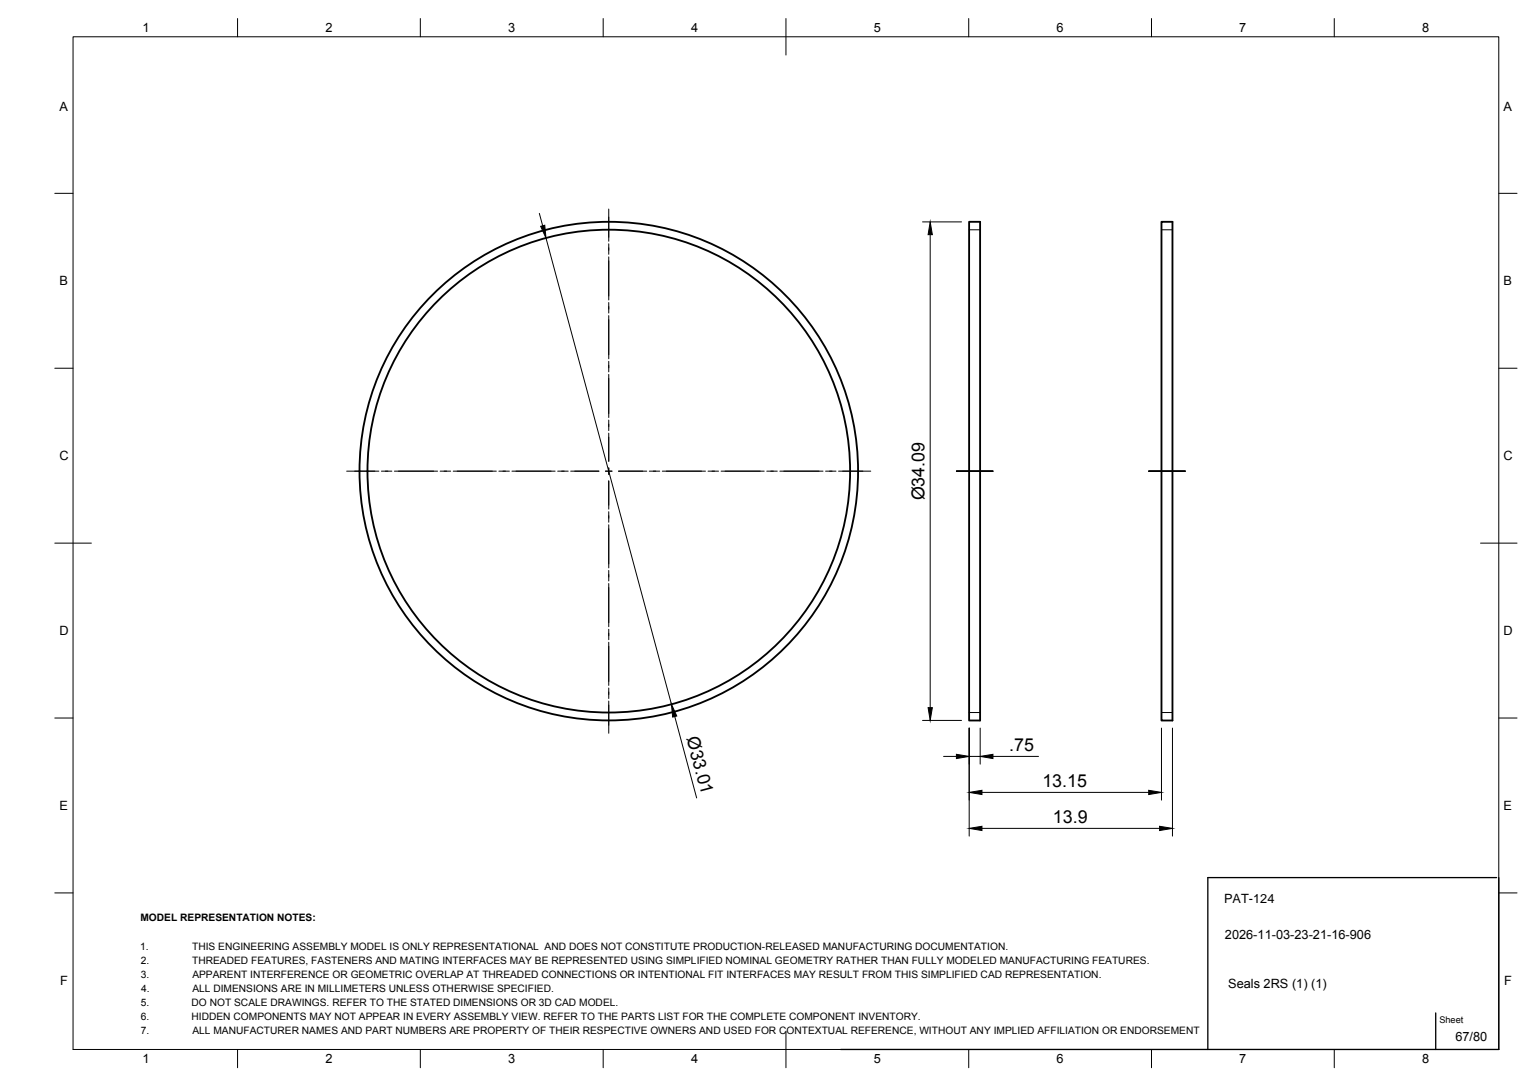
ISO-10303-21;
HEADER;
/* Generated by software containing ST-Developer
 * from STEP Tools, Inc. (www.steptools.com) 
 */

FILE_DESCRIPTION(
/* description */ ('XY cross-slide table'),
/* implementation_level */ '2;1');

FILE_NAME(
/* name */ 'Seals 2RS (1) (1).step',
/* time_stamp */ '2026-10-28T03:22:46-07:00',
/* author */ (''),
/* organization */ (''),
/* preprocessor_version */ 'ST-DEVELOPER v20.2',
/* originating_system */ 'Autodesk Translation Framework v15.17.0.0',
/* authorisation */ '');

FILE_SCHEMA (('AUTOMOTIVE_DESIGN { 1 0 10303 214 3 1 1 }'));
ENDSEC;

DATA;
#10=MECHANICAL_DESIGN_GEOMETRIC_PRESENTATION_REPRESENTATION('',(#1759,#1760),#62984);
#1564=SHAPE_REPRESENTATION_RELATIONSHIP('SRR','None',#63421,#1647);
#1647=ADVANCED_BREP_SHAPE_REPRESENTATION('',(#1868,#1869),#62958);
#1759=STYLED_ITEM('',(#63919),#1868);
#1760=STYLED_ITEM('',(#63919),#1869);
#1868=MANIFOLD_SOLID_BREP('Body1',#23057);
#1869=MANIFOLD_SOLID_BREP('Body2',#23058);
#2215=FACE_BOUND('',#5409,.T.);
#2216=FACE_BOUND('',#5412,.T.);
#2217=FACE_BOUND('',#5415,.T.);
#2218=FACE_BOUND('',#5418,.T.);
#2691=PLANE('',#25771);
#2692=PLANE('',#25776);
#2693=PLANE('',#25779);
#2694=PLANE('',#25784);
#3766=FACE_OUTER_BOUND('',#5408,.T.);
#3767=FACE_OUTER_BOUND('',#5410,.T.);
#3768=FACE_OUTER_BOUND('',#5411,.T.);
#3769=FACE_OUTER_BOUND('',#5413,.T.);
#3770=FACE_OUTER_BOUND('',#5414,.T.);
#3771=FACE_OUTER_BOUND('',#5416,.T.);
#3772=FACE_OUTER_BOUND('',#5417,.T.);
#3773=FACE_OUTER_BOUND('',#5419,.T.);
#5408=EDGE_LOOP('',(#19014));
#5409=EDGE_LOOP('',(#19015));
#5410=EDGE_LOOP('',(#19016,#19017,#19018,#19019));
#5411=EDGE_LOOP('',(#19020));
#5412=EDGE_LOOP('',(#19021));
#5413=EDGE_LOOP('',(#19022,#19023,#19024,#19025));
#5414=EDGE_LOOP('',(#19026));
#5415=EDGE_LOOP('',(#19027));
#5416=EDGE_LOOP('',(#19028,#19029,#19030,#19031));
#5417=EDGE_LOOP('',(#19032));
#5418=EDGE_LOOP('',(#19033));
#5419=EDGE_LOOP('',(#19034,#19035,#19036,#19037));
#6865=LINE('',#49619,#8352);
#6866=LINE('',#49624,#8353);
#6867=LINE('',#49633,#8354);
#6868=LINE('',#49638,#8355);
#8352=VECTOR('',#30972,1.70469);
#8353=VECTOR('',#30979,1.65031);
#8354=VECTOR('',#30990,1.70469);
#8355=VECTOR('',#30997,1.65031);
#9600=CIRCLE('',#25772,1.70469);
#9601=CIRCLE('',#25773,1.65031);
#9602=CIRCLE('',#25775,1.70469);
#9603=CIRCLE('',#25777,1.65031);
#9604=CIRCLE('',#25780,1.70469);
#9605=CIRCLE('',#25781,1.65031);
#9606=CIRCLE('',#25783,1.70469);
#9607=CIRCLE('',#25785,1.65031);
#11167=VERTEX_POINT('',#49612);
#11168=VERTEX_POINT('',#49614);
#11169=VERTEX_POINT('',#49617);
#11170=VERTEX_POINT('',#49621);
#11171=VERTEX_POINT('',#49626);
#11172=VERTEX_POINT('',#49628);
#11173=VERTEX_POINT('',#49631);
#11174=VERTEX_POINT('',#49635);
#13891=EDGE_CURVE('',#11167,#11167,#9600,.T.);
#13892=EDGE_CURVE('',#11168,#11168,#9601,.T.);
#13893=EDGE_CURVE('',#11169,#11169,#9602,.T.);
#13894=EDGE_CURVE('',#11169,#11167,#6865,.T.);
#13895=EDGE_CURVE('',#11170,#11170,#9603,.T.);
#13896=EDGE_CURVE('',#11170,#11168,#6866,.T.);
#13897=EDGE_CURVE('',#11171,#11171,#9604,.T.);
#13898=EDGE_CURVE('',#11172,#11172,#9605,.T.);
#13899=EDGE_CURVE('',#11173,#11173,#9606,.T.);
#13900=EDGE_CURVE('',#11173,#11171,#6867,.T.);
#13901=EDGE_CURVE('',#11174,#11174,#9607,.T.);
#13902=EDGE_CURVE('',#11174,#11172,#6868,.T.);
#19014=ORIENTED_EDGE('',*,*,#13891,.F.);
#19015=ORIENTED_EDGE('',*,*,#13892,.T.);
#19016=ORIENTED_EDGE('',*,*,#13893,.F.);
#19017=ORIENTED_EDGE('',*,*,#13894,.T.);
#19018=ORIENTED_EDGE('',*,*,#13891,.T.);
#19019=ORIENTED_EDGE('',*,*,#13894,.F.);
#19020=ORIENTED_EDGE('',*,*,#13893,.T.);
#19021=ORIENTED_EDGE('',*,*,#13895,.F.);
#19022=ORIENTED_EDGE('',*,*,#13895,.T.);
#19023=ORIENTED_EDGE('',*,*,#13896,.T.);
#19024=ORIENTED_EDGE('',*,*,#13892,.F.);
#19025=ORIENTED_EDGE('',*,*,#13896,.F.);
#19026=ORIENTED_EDGE('',*,*,#13897,.F.);
#19027=ORIENTED_EDGE('',*,*,#13898,.T.);
#19028=ORIENTED_EDGE('',*,*,#13899,.F.);
#19029=ORIENTED_EDGE('',*,*,#13900,.T.);
#19030=ORIENTED_EDGE('',*,*,#13897,.T.);
#19031=ORIENTED_EDGE('',*,*,#13900,.F.);
#19032=ORIENTED_EDGE('',*,*,#13899,.T.);
#19033=ORIENTED_EDGE('',*,*,#13901,.F.);
#19034=ORIENTED_EDGE('',*,*,#13901,.T.);
#19035=ORIENTED_EDGE('',*,*,#13902,.T.);
#19036=ORIENTED_EDGE('',*,*,#13898,.F.);
#19037=ORIENTED_EDGE('',*,*,#13902,.F.);
#21436=CYLINDRICAL_SURFACE('',#25774,1.70469);
#21437=CYLINDRICAL_SURFACE('',#25778,1.65031);
#21438=CYLINDRICAL_SURFACE('',#25782,1.70469);
#21439=CYLINDRICAL_SURFACE('',#25786,1.65031);
#22547=ADVANCED_FACE('',(#3766,#2215),#2691,.T.);
#22548=ADVANCED_FACE('',(#3767),#21436,.T.);
#22549=ADVANCED_FACE('',(#3768,#2216),#2692,.T.);
#22550=ADVANCED_FACE('',(#3769),#21437,.F.);
#22551=ADVANCED_FACE('',(#3770,#2217),#2693,.T.);
#22552=ADVANCED_FACE('',(#3771),#21438,.T.);
#22553=ADVANCED_FACE('',(#3772,#2218),#2694,.T.);
#22554=ADVANCED_FACE('',(#3773),#21439,.F.);
#23057=CLOSED_SHELL('',(#22547,#22548,#22549,#22550));
#23058=CLOSED_SHELL('',(#22551,#22552,#22553,#22554));
#25770=AXIS2_PLACEMENT_3D('',#49610,#30960,#30961);
#25771=AXIS2_PLACEMENT_3D('',#49611,#30962,#30963);
#25772=AXIS2_PLACEMENT_3D('',#49613,#30964,#30965);
#25773=AXIS2_PLACEMENT_3D('',#49615,#30966,#30967);
#25774=AXIS2_PLACEMENT_3D('',#49616,#30968,#30969);
#25775=AXIS2_PLACEMENT_3D('',#49618,#30970,#30971);
#25776=AXIS2_PLACEMENT_3D('',#49620,#30973,#30974);
#25777=AXIS2_PLACEMENT_3D('',#49622,#30975,#30976);
#25778=AXIS2_PLACEMENT_3D('',#49623,#30977,#30978);
#25779=AXIS2_PLACEMENT_3D('',#49625,#30980,#30981);
#25780=AXIS2_PLACEMENT_3D('',#49627,#30982,#30983);
#25781=AXIS2_PLACEMENT_3D('',#49629,#30984,#30985);
#25782=AXIS2_PLACEMENT_3D('',#49630,#30986,#30987);
#25783=AXIS2_PLACEMENT_3D('',#49632,#30988,#30989);
#25784=AXIS2_PLACEMENT_3D('',#49634,#30991,#30992);
#25785=AXIS2_PLACEMENT_3D('',#49636,#30993,#30994);
#25786=AXIS2_PLACEMENT_3D('',#49637,#30995,#30996);
#30960=DIRECTION('axis',(0.,0.,1.));
#30961=DIRECTION('refdir',(1.,0.,0.));
#30962=DIRECTION('center_axis',(0.,1.,0.));
#30963=DIRECTION('ref_axis',(0.,0.,1.));
#30964=DIRECTION('center_axis',(0.,-1.,0.));
#30965=DIRECTION('ref_axis',(1.,0.,0.));
#30966=DIRECTION('center_axis',(0.,-1.,0.));
#30967=DIRECTION('ref_axis',(1.,0.,0.));
#30968=DIRECTION('center_axis',(0.,-1.,0.));
#30969=DIRECTION('ref_axis',(1.,0.,0.));
#30970=DIRECTION('center_axis',(0.,-1.,0.));
#30971=DIRECTION('ref_axis',(1.,0.,0.));
#30972=DIRECTION('',(0.,1.,0.));
#30973=DIRECTION('center_axis',(0.,-1.,0.));
#30974=DIRECTION('ref_axis',(0.,0.,-1.));
#30975=DIRECTION('center_axis',(0.,-1.,0.));
#30976=DIRECTION('ref_axis',(1.,0.,0.));
#30977=DIRECTION('center_axis',(0.,-1.,0.));
#30978=DIRECTION('ref_axis',(1.,0.,0.));
#30979=DIRECTION('',(0.,1.,0.));
#30980=DIRECTION('center_axis',(0.,1.,0.));
#30981=DIRECTION('ref_axis',(0.,0.,1.));
#30982=DIRECTION('center_axis',(0.,-1.,0.));
#30983=DIRECTION('ref_axis',(1.,0.,0.));
#30984=DIRECTION('center_axis',(0.,-1.,0.));
#30985=DIRECTION('ref_axis',(1.,0.,0.));
#30986=DIRECTION('center_axis',(0.,-1.,0.));
#30987=DIRECTION('ref_axis',(1.,0.,0.));
#30988=DIRECTION('center_axis',(0.,-1.,0.));
#30989=DIRECTION('ref_axis',(1.,0.,0.));
#30990=DIRECTION('',(0.,1.,0.));
#30991=DIRECTION('center_axis',(0.,-1.,0.));
#30992=DIRECTION('ref_axis',(0.,0.,-1.));
#30993=DIRECTION('center_axis',(0.,-1.,0.));
#30994=DIRECTION('ref_axis',(1.,0.,0.));
#30995=DIRECTION('center_axis',(0.,-1.,0.));
#30996=DIRECTION('ref_axis',(1.,0.,0.));
#30997=DIRECTION('',(0.,1.,0.));
#49610=CARTESIAN_POINT('',(0.,0.,0.));
#49611=CARTESIAN_POINT('Origin',(1.70469,0.695,0.));
#49612=CARTESIAN_POINT('',(-1.70469,0.695,-2.0876431520385E-16));
#49613=CARTESIAN_POINT('Origin',(0.,0.695,0.));
#49614=CARTESIAN_POINT('',(-1.65031,0.695,-2.02104685910087E-16));
#49615=CARTESIAN_POINT('Origin',(0.,0.695,0.));
#49616=CARTESIAN_POINT('Origin',(0.,0.6575,0.));
#49617=CARTESIAN_POINT('',(-1.70469,0.62,-2.0876431520385E-16));
#49618=CARTESIAN_POINT('Origin',(0.,0.62,0.));
#49619=CARTESIAN_POINT('',(-1.70469,0.6575,-2.0876431520385E-16));
#49620=CARTESIAN_POINT('Origin',(1.65031,0.62,0.));
#49621=CARTESIAN_POINT('',(-1.65031,0.62,-2.02104685910087E-16));
#49622=CARTESIAN_POINT('Origin',(0.,0.62,0.));
#49623=CARTESIAN_POINT('Origin',(0.,0.6575,0.));
#49624=CARTESIAN_POINT('',(-1.65031,0.6575,-2.02104685910087E-16));
#49625=CARTESIAN_POINT('Origin',(1.70469,-0.62,0.));
#49626=CARTESIAN_POINT('',(-1.70469,-0.62,-2.0876431520385E-16));
#49627=CARTESIAN_POINT('Origin',(0.,-0.62,0.));
#49628=CARTESIAN_POINT('',(-1.65031,-0.62,-2.02104685910087E-16));
#49629=CARTESIAN_POINT('Origin',(0.,-0.62,0.));
#49630=CARTESIAN_POINT('Origin',(0.,-0.6575,0.));
#49631=CARTESIAN_POINT('',(-1.70469,-0.695,-2.0876431520385E-16));
#49632=CARTESIAN_POINT('Origin',(0.,-0.695,0.));
#49633=CARTESIAN_POINT('',(-1.70469,-0.6575,-2.0876431520385E-16));
#49634=CARTESIAN_POINT('Origin',(1.65031,-0.695,0.));
#49635=CARTESIAN_POINT('',(-1.65031,-0.695,-2.02104685910087E-16));
#49636=CARTESIAN_POINT('Origin',(0.,-0.695,0.));
#49637=CARTESIAN_POINT('Origin',(0.,-0.6575,0.));
#49638=CARTESIAN_POINT('',(-1.65031,-0.6575,-2.02104685910087E-16));
#62859=UNCERTAINTY_MEASURE_WITH_UNIT(LENGTH_MEASURE(0.001),#62985,
'DISTANCE_ACCURACY_VALUE',
'Maximum model space distance between geometric entities at asserted c
onnectivities');
#62885=UNCERTAINTY_MEASURE_WITH_UNIT(LENGTH_MEASURE(0.001),#62985,
'DISTANCE_ACCURACY_VALUE',
'Maximum model space distance between geometric entities at asserted c
onnectivities');
#62958=(
GEOMETRIC_REPRESENTATION_CONTEXT(3)
GLOBAL_UNCERTAINTY_ASSIGNED_CONTEXT((#62859))
GLOBAL_UNIT_ASSIGNED_CONTEXT((#62985,#62987,#62988))
REPRESENTATION_CONTEXT('','3D')
);
#62984=(
GEOMETRIC_REPRESENTATION_CONTEXT(3)
GLOBAL_UNCERTAINTY_ASSIGNED_CONTEXT((#62885))
GLOBAL_UNIT_ASSIGNED_CONTEXT((#62985,#62987,#62988))
REPRESENTATION_CONTEXT('','3D')
);
#62985=(
LENGTH_UNIT()
NAMED_UNIT(*)
SI_UNIT(.CENTI.,.METRE.)
);
#62987=(
NAMED_UNIT(*)
PLANE_ANGLE_UNIT()
SI_UNIT($,.RADIAN.)
);
#62988=(
NAMED_UNIT(*)
SI_UNIT($,.STERADIAN.)
SOLID_ANGLE_UNIT()
);
#63061=SHAPE_DEFINITION_REPRESENTATION(#63244,#63421);
#63244=PRODUCT_DEFINITION_SHAPE('',$,#63520);
#63421=SHAPE_REPRESENTATION('',(#25770),#62958);
#63447=PRODUCT_DEFINITION_CONTEXT('part definition',#63743,'design');
#63520=PRODUCT_DEFINITION('Seals 2RS (1) (1)','Seals 2RS (1) (1)',#63618,#63447);
#63618=PRODUCT_DEFINITION_FORMATION('',$,#63817);
#63743=APPLICATION_CONTEXT(
'Core Data for Automotive Mechanical Design Process');
#63744=PRODUCT_CONTEXT('part definition',#63743,'mechanical');
#63817=PRODUCT('Seals 2RS (1) (1)','Seals 2RS (1) (1)','Seals 2RS (1) (1)',(#63744));
#63913=COLOUR_RGB('Black',0.12,0.14,0.17);
#63914=FILL_AREA_STYLE_COLOUR('',#63913);
#63915=FILL_AREA_STYLE('',(#63914));
#63916=SURFACE_STYLE_FILL_AREA(#63915);
#63917=SURFACE_SIDE_STYLE('',(#63916));
#63918=SURFACE_STYLE_USAGE(.BOTH.,#63917);
#63919=PRESENTATION_STYLE_ASSIGNMENT((#63918));
ENDSEC;
END-ISO-10303-21;
